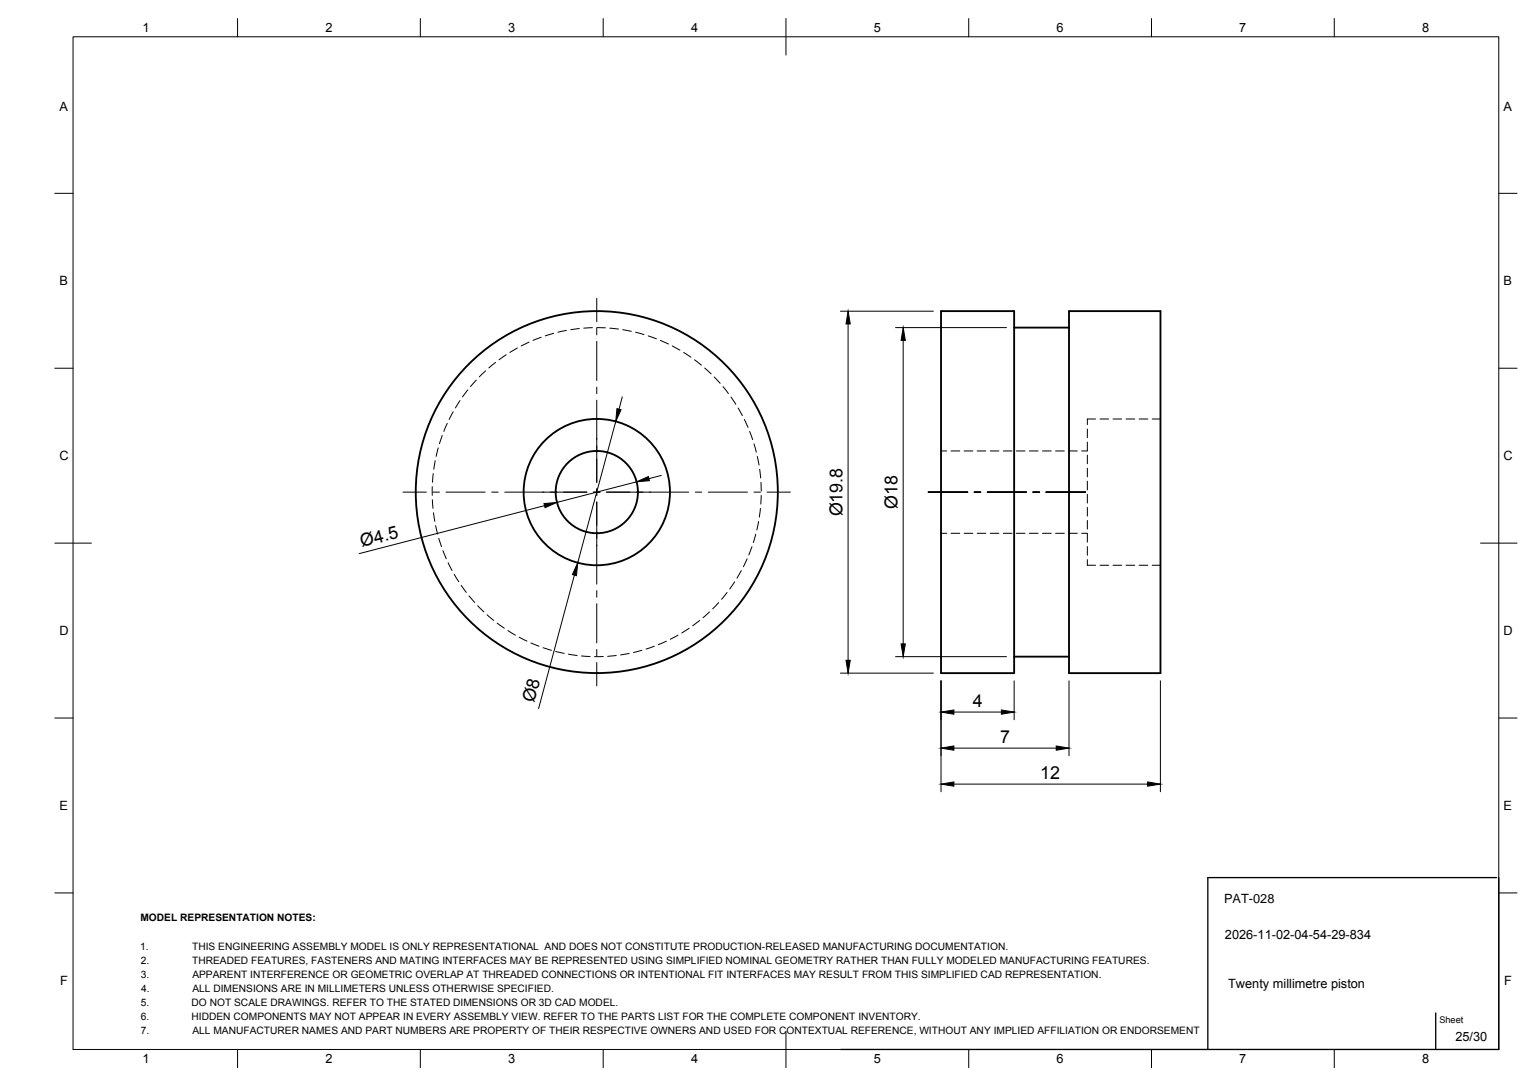
ISO-10303-21;
HEADER;
/* Generated by software containing ST-Developer
 * from STEP Tools, Inc. (www.steptools.com) 
 */

FILE_DESCRIPTION(
/* description */ ('Cylinder foot and clevis mount kit'),
/* implementation_level */ '2;1');

FILE_NAME(
/* name */ 'Twenty millimetre piston.step',
/* time_stamp */ '2026-10-27T20:10:43-07:00',
/* author */ (''),
/* organization */ (''),
/* preprocessor_version */ 'ST-DEVELOPER v20.2',
/* originating_system */ 'Autodesk Translation Framework v15.17.0.0',
/* authorisation */ '');

FILE_SCHEMA (('AUTOMOTIVE_DESIGN { 1 0 10303 214 3 1 1 }'));
ENDSEC;

DATA;
#10=MECHANICAL_DESIGN_GEOMETRIC_PRESENTATION_REPRESENTATION('',(#357),#9102);
#301=SHAPE_REPRESENTATION_RELATIONSHIP('SRR','None',#9250,#329);
#329=ADVANCED_BREP_SHAPE_REPRESENTATION('',(#384),#9093);
#357=STYLED_ITEM('',(#9474),#384);
#384=MANIFOLD_SOLID_BREP('Body1',#4944);
#474=FACE_BOUND('',#1313,.T.);
#475=FACE_BOUND('',#1316,.T.);
#476=FACE_BOUND('',#1318,.T.);
#477=FACE_BOUND('',#1323,.T.);
#478=FACE_BOUND('',#1325,.T.);
#647=PLANE('',#5742);
#648=PLANE('',#5747);
#649=PLANE('',#5749);
#650=PLANE('',#5757);
#651=PLANE('',#5758);
#923=FACE_OUTER_BOUND('',#1311,.T.);
#924=FACE_OUTER_BOUND('',#1312,.T.);
#925=FACE_OUTER_BOUND('',#1314,.T.);
#926=FACE_OUTER_BOUND('',#1315,.T.);
#927=FACE_OUTER_BOUND('',#1317,.T.);
#928=FACE_OUTER_BOUND('',#1319,.T.);
#929=FACE_OUTER_BOUND('',#1320,.T.);
#930=FACE_OUTER_BOUND('',#1321,.T.);
#931=FACE_OUTER_BOUND('',#1322,.T.);
#932=FACE_OUTER_BOUND('',#1324,.T.);
#1311=EDGE_LOOP('',(#4209,#4210,#4211,#4212));
#1312=EDGE_LOOP('',(#4213));
#1313=EDGE_LOOP('',(#4214));
#1314=EDGE_LOOP('',(#4215,#4216,#4217,#4218));
#1315=EDGE_LOOP('',(#4219));
#1316=EDGE_LOOP('',(#4220));
#1317=EDGE_LOOP('',(#4221));
#1318=EDGE_LOOP('',(#4222));
#1319=EDGE_LOOP('',(#4223,#4224,#4225,#4226));
#1320=EDGE_LOOP('',(#4227,#4228,#4229,#4230));
#1321=EDGE_LOOP('',(#4231,#4232,#4233,#4234));
#1322=EDGE_LOOP('',(#4235));
#1323=EDGE_LOOP('',(#4236));
#1324=EDGE_LOOP('',(#4237));
#1325=EDGE_LOOP('',(#4238));
#1664=LINE('',#8549,#2013);
#1665=LINE('',#8558,#2014);
#1666=LINE('',#8568,#2015);
#1667=LINE('',#8572,#2016);
#1668=LINE('',#8577,#2017);
#2013=VECTOR('',#7101,0.4);
#2014=VECTOR('',#7112,0.9);
#2015=VECTOR('',#7125,0.99);
#2016=VECTOR('',#7130,0.225);
#2017=VECTOR('',#7137,0.99);
#2275=CIRCLE('',#5740,0.4);
#2276=CIRCLE('',#5741,0.4);
#2277=CIRCLE('',#5743,0.225);
#2278=CIRCLE('',#5745,0.9);
#2279=CIRCLE('',#5746,0.9);
#2280=CIRCLE('',#5748,0.99);
#2281=CIRCLE('',#5750,0.99);
#2282=CIRCLE('',#5752,0.99);
#2283=CIRCLE('',#5754,0.225);
#2284=CIRCLE('',#5756,0.99);
#2611=VERTEX_POINT('',#8546);
#2612=VERTEX_POINT('',#8548);
#2613=VERTEX_POINT('',#8552);
#2614=VERTEX_POINT('',#8555);
#2615=VERTEX_POINT('',#8557);
#2616=VERTEX_POINT('',#8561);
#2617=VERTEX_POINT('',#8564);
#2618=VERTEX_POINT('',#8567);
#2619=VERTEX_POINT('',#8571);
#2620=VERTEX_POINT('',#8575);
#3159=EDGE_CURVE('',#2611,#2611,#2275,.T.);
#3160=EDGE_CURVE('',#2611,#2612,#1664,.T.);
#3161=EDGE_CURVE('',#2612,#2612,#2276,.T.);
#3162=EDGE_CURVE('',#2613,#2613,#2277,.T.);
#3163=EDGE_CURVE('',#2614,#2614,#2278,.T.);
#3164=EDGE_CURVE('',#2614,#2615,#1665,.T.);
#3165=EDGE_CURVE('',#2615,#2615,#2279,.T.);
#3166=EDGE_CURVE('',#2616,#2616,#2280,.T.);
#3167=EDGE_CURVE('',#2617,#2617,#2281,.T.);
#3168=EDGE_CURVE('',#2617,#2618,#1666,.T.);
#3169=EDGE_CURVE('',#2618,#2618,#2282,.T.);
#3170=EDGE_CURVE('',#2613,#2619,#1667,.T.);
#3171=EDGE_CURVE('',#2619,#2619,#2283,.T.);
#3172=EDGE_CURVE('',#2620,#2620,#2284,.T.);
#3173=EDGE_CURVE('',#2620,#2616,#1668,.T.);
#4209=ORIENTED_EDGE('',*,*,#3159,.F.);
#4210=ORIENTED_EDGE('',*,*,#3160,.T.);
#4211=ORIENTED_EDGE('',*,*,#3161,.F.);
#4212=ORIENTED_EDGE('',*,*,#3160,.F.);
#4213=ORIENTED_EDGE('',*,*,#3159,.T.);
#4214=ORIENTED_EDGE('',*,*,#3162,.F.);
#4215=ORIENTED_EDGE('',*,*,#3163,.F.);
#4216=ORIENTED_EDGE('',*,*,#3164,.T.);
#4217=ORIENTED_EDGE('',*,*,#3165,.T.);
#4218=ORIENTED_EDGE('',*,*,#3164,.F.);
#4219=ORIENTED_EDGE('',*,*,#3166,.F.);
#4220=ORIENTED_EDGE('',*,*,#3165,.F.);
#4221=ORIENTED_EDGE('',*,*,#3167,.F.);
#4222=ORIENTED_EDGE('',*,*,#3163,.T.);
#4223=ORIENTED_EDGE('',*,*,#3167,.T.);
#4224=ORIENTED_EDGE('',*,*,#3168,.T.);
#4225=ORIENTED_EDGE('',*,*,#3169,.T.);
#4226=ORIENTED_EDGE('',*,*,#3168,.F.);
#4227=ORIENTED_EDGE('',*,*,#3162,.T.);
#4228=ORIENTED_EDGE('',*,*,#3170,.T.);
#4229=ORIENTED_EDGE('',*,*,#3171,.T.);
#4230=ORIENTED_EDGE('',*,*,#3170,.F.);
#4231=ORIENTED_EDGE('',*,*,#3172,.F.);
#4232=ORIENTED_EDGE('',*,*,#3173,.T.);
#4233=ORIENTED_EDGE('',*,*,#3166,.T.);
#4234=ORIENTED_EDGE('',*,*,#3173,.F.);
#4235=ORIENTED_EDGE('',*,*,#3172,.T.);
#4236=ORIENTED_EDGE('',*,*,#3161,.T.);
#4237=ORIENTED_EDGE('',*,*,#3169,.F.);
#4238=ORIENTED_EDGE('',*,*,#3171,.F.);
#4598=CYLINDRICAL_SURFACE('',#5739,0.4);
#4599=CYLINDRICAL_SURFACE('',#5744,0.9);
#4600=CYLINDRICAL_SURFACE('',#5751,0.99);
#4601=CYLINDRICAL_SURFACE('',#5753,0.225);
#4602=CYLINDRICAL_SURFACE('',#5755,0.99);
#4846=ADVANCED_FACE('',(#923),#4598,.F.);
#4847=ADVANCED_FACE('',(#924,#474),#647,.T.);
#4848=ADVANCED_FACE('',(#925),#4599,.T.);
#4849=ADVANCED_FACE('',(#926,#475),#648,.F.);
#4850=ADVANCED_FACE('',(#927,#476),#649,.T.);
#4851=ADVANCED_FACE('',(#928),#4600,.T.);
#4852=ADVANCED_FACE('',(#929),#4601,.F.);
#4853=ADVANCED_FACE('',(#930),#4602,.T.);
#4854=ADVANCED_FACE('',(#931,#477),#650,.T.);
#4855=ADVANCED_FACE('',(#932,#478),#651,.F.);
#4944=CLOSED_SHELL('',(#4846,#4847,#4848,#4849,#4850,#4851,#4852,#4853,
#4854,#4855));
#5738=AXIS2_PLACEMENT_3D('',#8544,#7095,#7096);
#5739=AXIS2_PLACEMENT_3D('',#8545,#7097,#7098);
#5740=AXIS2_PLACEMENT_3D('',#8547,#7099,#7100);
#5741=AXIS2_PLACEMENT_3D('',#8550,#7102,#7103);
#5742=AXIS2_PLACEMENT_3D('',#8551,#7104,#7105);
#5743=AXIS2_PLACEMENT_3D('',#8553,#7106,#7107);
#5744=AXIS2_PLACEMENT_3D('',#8554,#7108,#7109);
#5745=AXIS2_PLACEMENT_3D('',#8556,#7110,#7111);
#5746=AXIS2_PLACEMENT_3D('',#8559,#7113,#7114);
#5747=AXIS2_PLACEMENT_3D('',#8560,#7115,#7116);
#5748=AXIS2_PLACEMENT_3D('',#8562,#7117,#7118);
#5749=AXIS2_PLACEMENT_3D('',#8563,#7119,#7120);
#5750=AXIS2_PLACEMENT_3D('',#8565,#7121,#7122);
#5751=AXIS2_PLACEMENT_3D('',#8566,#7123,#7124);
#5752=AXIS2_PLACEMENT_3D('',#8569,#7126,#7127);
#5753=AXIS2_PLACEMENT_3D('',#8570,#7128,#7129);
#5754=AXIS2_PLACEMENT_3D('',#8573,#7131,#7132);
#5755=AXIS2_PLACEMENT_3D('',#8574,#7133,#7134);
#5756=AXIS2_PLACEMENT_3D('',#8576,#7135,#7136);
#5757=AXIS2_PLACEMENT_3D('',#8578,#7138,#7139);
#5758=AXIS2_PLACEMENT_3D('',#8579,#7140,#7141);
#7095=DIRECTION('axis',(0.,0.,1.));
#7096=DIRECTION('refdir',(1.,0.,0.));
#7097=DIRECTION('center_axis',(0.,1.,0.));
#7098=DIRECTION('ref_axis',(1.,0.,0.));
#7099=DIRECTION('center_axis',(0.,1.,0.));
#7100=DIRECTION('ref_axis',(1.,0.,0.));
#7101=DIRECTION('',(0.,1.,0.));
#7102=DIRECTION('center_axis',(0.,-1.,0.));
#7103=DIRECTION('ref_axis',(1.,0.,0.));
#7104=DIRECTION('center_axis',(0.,1.,0.));
#7105=DIRECTION('ref_axis',(1.,0.,0.));
#7106=DIRECTION('center_axis',(0.,1.,0.));
#7107=DIRECTION('ref_axis',(1.,0.,0.));
#7108=DIRECTION('center_axis',(0.,1.,0.));
#7109=DIRECTION('ref_axis',(1.,0.,0.));
#7110=DIRECTION('center_axis',(0.,-1.,0.));
#7111=DIRECTION('ref_axis',(1.,0.,0.));
#7112=DIRECTION('',(0.,1.,0.));
#7113=DIRECTION('center_axis',(0.,-1.,0.));
#7114=DIRECTION('ref_axis',(1.,0.,0.));
#7115=DIRECTION('center_axis',(0.,1.,0.));
#7116=DIRECTION('ref_axis',(1.,0.,0.));
#7117=DIRECTION('center_axis',(0.,1.,0.));
#7118=DIRECTION('ref_axis',(1.,0.,0.));
#7119=DIRECTION('center_axis',(0.,1.,0.));
#7120=DIRECTION('ref_axis',(1.,0.,0.));
#7121=DIRECTION('center_axis',(0.,-1.,0.));
#7122=DIRECTION('ref_axis',(1.,0.,0.));
#7123=DIRECTION('center_axis',(0.,1.,0.));
#7124=DIRECTION('ref_axis',(1.,0.,0.));
#7125=DIRECTION('',(0.,-1.,0.));
#7126=DIRECTION('center_axis',(0.,1.,0.));
#7127=DIRECTION('ref_axis',(1.,0.,0.));
#7128=DIRECTION('center_axis',(0.,1.,0.));
#7129=DIRECTION('ref_axis',(1.,0.,0.));
#7130=DIRECTION('',(0.,-1.,0.));
#7131=DIRECTION('center_axis',(0.,-1.,0.));
#7132=DIRECTION('ref_axis',(1.,0.,0.));
#7133=DIRECTION('center_axis',(0.,1.,0.));
#7134=DIRECTION('ref_axis',(1.,0.,0.));
#7135=DIRECTION('center_axis',(0.,1.,0.));
#7136=DIRECTION('ref_axis',(1.,0.,0.));
#7137=DIRECTION('',(0.,-1.,0.));
#7138=DIRECTION('center_axis',(0.,1.,0.));
#7139=DIRECTION('ref_axis',(1.,0.,0.));
#7140=DIRECTION('center_axis',(0.,1.,0.));
#7141=DIRECTION('ref_axis',(1.,0.,0.));
#8544=CARTESIAN_POINT('',(0.,0.,0.));
#8545=CARTESIAN_POINT('Origin',(0.,3.2,4.5));
#8546=CARTESIAN_POINT('',(-0.4,3.2,4.5));
#8547=CARTESIAN_POINT('Origin',(0.,3.2,4.5));
#8548=CARTESIAN_POINT('',(-0.4,3.6,4.5));
#8549=CARTESIAN_POINT('',(-0.4,3.2,4.5));
#8550=CARTESIAN_POINT('Origin',(0.,3.6,4.5));
#8551=CARTESIAN_POINT('Origin',(0.,3.2,4.5));
#8552=CARTESIAN_POINT('',(-0.225,3.2,4.5));
#8553=CARTESIAN_POINT('Origin',(0.,3.2,4.5));
#8554=CARTESIAN_POINT('Origin',(0.,2.8,4.5));
#8555=CARTESIAN_POINT('',(-0.9,2.8,4.5));
#8556=CARTESIAN_POINT('Origin',(0.,2.8,4.5));
#8557=CARTESIAN_POINT('',(-0.9,3.1,4.5));
#8558=CARTESIAN_POINT('',(-0.9,2.8,4.5));
#8559=CARTESIAN_POINT('Origin',(0.,3.1,4.5));
#8560=CARTESIAN_POINT('Origin',(0.,3.1,4.5));
#8561=CARTESIAN_POINT('',(-0.99,3.1,4.5));
#8562=CARTESIAN_POINT('Origin',(0.,3.1,4.5));
#8563=CARTESIAN_POINT('Origin',(0.,2.8,4.5));
#8564=CARTESIAN_POINT('',(-0.99,2.8,4.5));
#8565=CARTESIAN_POINT('Origin',(0.,2.8,4.5));
#8566=CARTESIAN_POINT('Origin',(0.,2.4,4.5));
#8567=CARTESIAN_POINT('',(-0.99,2.4,4.5));
#8568=CARTESIAN_POINT('',(-0.99,2.4,4.5));
#8569=CARTESIAN_POINT('Origin',(0.,2.4,4.5));
#8570=CARTESIAN_POINT('Origin',(0.,2.4,4.5));
#8571=CARTESIAN_POINT('',(-0.225,2.4,4.5));
#8572=CARTESIAN_POINT('',(-0.225,2.4,4.5));
#8573=CARTESIAN_POINT('Origin',(0.,2.4,4.5));
#8574=CARTESIAN_POINT('Origin',(0.,2.4,4.5));
#8575=CARTESIAN_POINT('',(-0.99,3.6,4.5));
#8576=CARTESIAN_POINT('Origin',(0.,3.6,4.5));
#8577=CARTESIAN_POINT('',(-0.99,2.4,4.5));
#8578=CARTESIAN_POINT('Origin',(0.,3.6,4.5));
#8579=CARTESIAN_POINT('Origin',(0.,2.4,4.5));
#9060=UNCERTAINTY_MEASURE_WITH_UNIT(LENGTH_MEASURE(0.001),#9103,
'DISTANCE_ACCURACY_VALUE',
'Maximum model space distance between geometric entities at asserted c
onnectivities');
#9069=UNCERTAINTY_MEASURE_WITH_UNIT(LENGTH_MEASURE(0.001),#9103,
'DISTANCE_ACCURACY_VALUE',
'Maximum model space distance between geometric entities at asserted c
onnectivities');
#9093=(
GEOMETRIC_REPRESENTATION_CONTEXT(3)
GLOBAL_UNCERTAINTY_ASSIGNED_CONTEXT((#9060))
GLOBAL_UNIT_ASSIGNED_CONTEXT((#9103,#9105,#9106))
REPRESENTATION_CONTEXT('','3D')
);
#9102=(
GEOMETRIC_REPRESENTATION_CONTEXT(3)
GLOBAL_UNCERTAINTY_ASSIGNED_CONTEXT((#9069))
GLOBAL_UNIT_ASSIGNED_CONTEXT((#9103,#9105,#9106))
REPRESENTATION_CONTEXT('','3D')
);
#9103=(
LENGTH_UNIT()
NAMED_UNIT(*)
SI_UNIT(.CENTI.,.METRE.)
);
#9105=(
NAMED_UNIT(*)
PLANE_ANGLE_UNIT()
SI_UNIT($,.RADIAN.)
);
#9106=(
NAMED_UNIT(*)
SI_UNIT($,.STERADIAN.)
SOLID_ANGLE_UNIT()
);
#9130=SHAPE_DEFINITION_REPRESENTATION(#9205,#9250);
#9205=PRODUCT_DEFINITION_SHAPE('',$,#9283);
#9250=SHAPE_REPRESENTATION('',(#5738),#9093);
#9259=PRODUCT_DEFINITION_CONTEXT('part definition',#9357,'design');
#9283=PRODUCT_DEFINITION('Twenty millimetre piston',
'Twenty millimetre piston',#9315,#9259);
#9315=PRODUCT_DEFINITION_FORMATION('',$,#9382);
#9357=APPLICATION_CONTEXT(
'Core Data for Automotive Mechanical Design Process');
#9358=PRODUCT_CONTEXT('part definition',#9357,'mechanical');
#9382=PRODUCT('Twenty millimetre piston','Twenty millimetre piston',
'Twenty millimetre piston',(#9358));
#9468=COLOUR_RGB('Off White',0.89,0.88,0.83);
#9469=FILL_AREA_STYLE_COLOUR('',#9468);
#9470=FILL_AREA_STYLE('',(#9469));
#9471=SURFACE_STYLE_FILL_AREA(#9470);
#9472=SURFACE_SIDE_STYLE('',(#9471));
#9473=SURFACE_STYLE_USAGE(.BOTH.,#9472);
#9474=PRESENTATION_STYLE_ASSIGNMENT((#9473));
ENDSEC;
END-ISO-10303-21;
